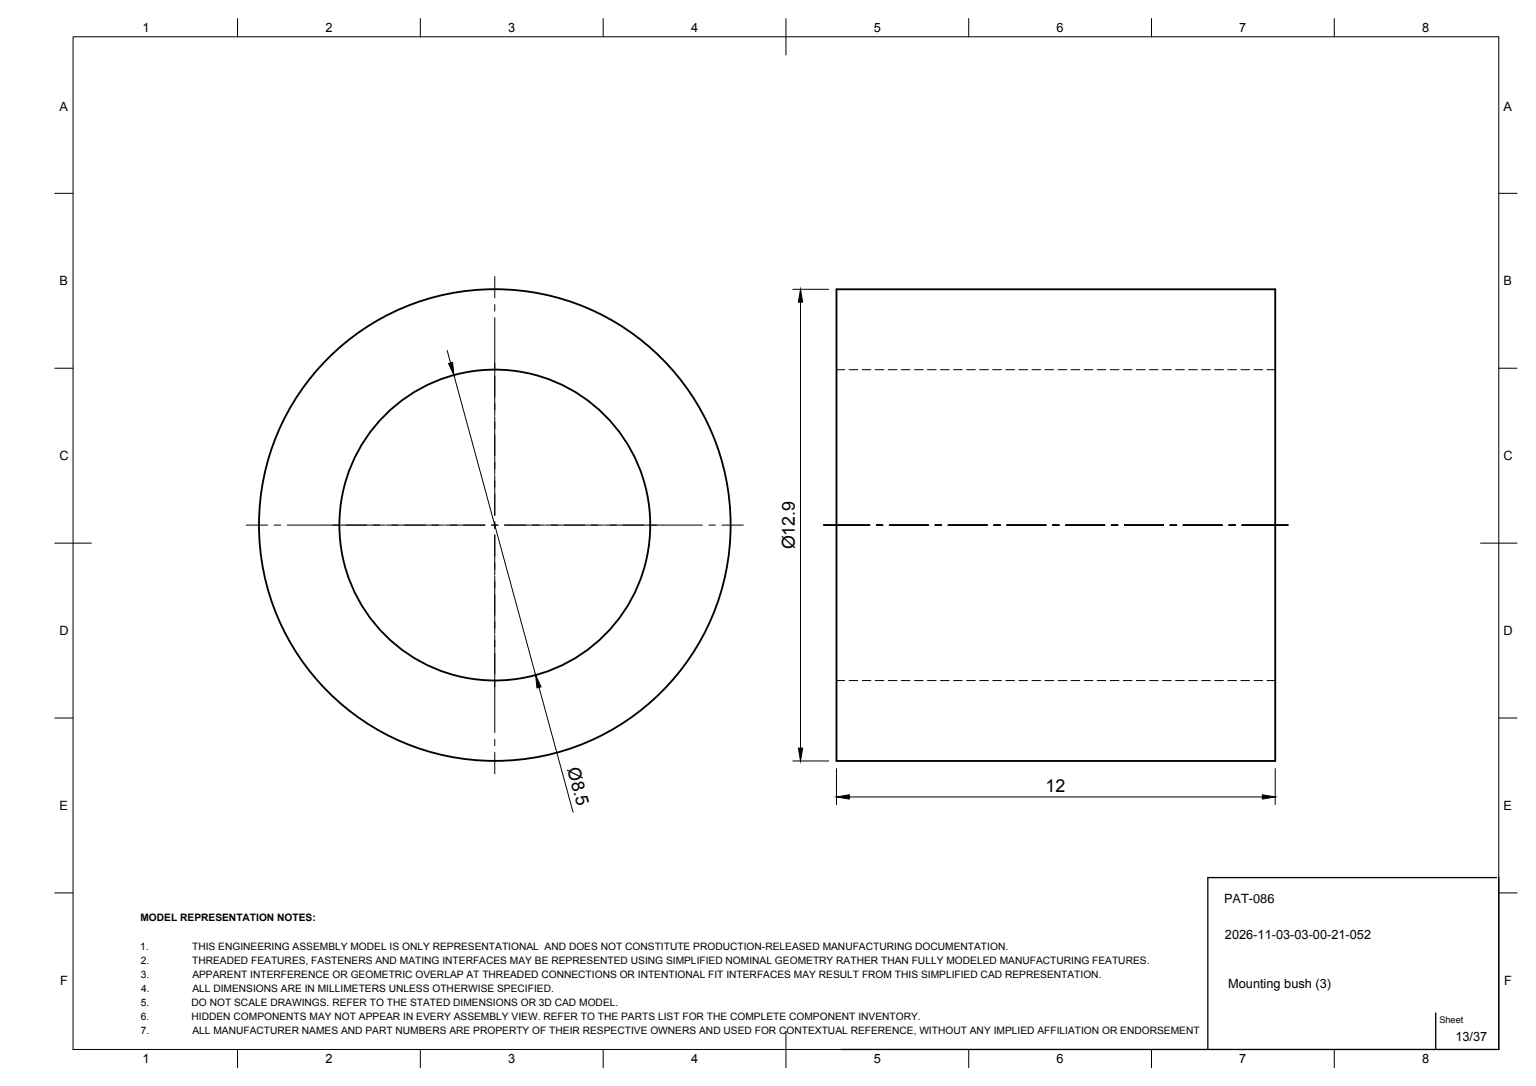
ISO-10303-21;
HEADER;
/* Generated by software containing ST-Developer
 * from STEP Tools, Inc. (www.steptools.com) 
 */

FILE_DESCRIPTION(
/* description */ ('Ratchet and pawl hand winch drum'),
/* implementation_level */ '2;1');

FILE_NAME(
/* name */ 'Mounting bush (3).step',
/* time_stamp */ '2026-10-27T12:42:58-07:00',
/* author */ (''),
/* organization */ (''),
/* preprocessor_version */ 'ST-DEVELOPER v20.2',
/* originating_system */ 'Autodesk Translation Framework v15.17.0.0',
/* authorisation */ '');

FILE_SCHEMA (('AUTOMOTIVE_DESIGN { 1 0 10303 214 3 1 1 }'));
ENDSEC;

DATA;
#10=MECHANICAL_DESIGN_GEOMETRIC_PRESENTATION_REPRESENTATION('',(#397),#11801);
#329=SHAPE_REPRESENTATION_RELATIONSHIP('SRR','None',#11955,#363);
#363=ADVANCED_BREP_SHAPE_REPRESENTATION('',(#432),#11772);
#397=STYLED_ITEM('',(#12206),#432);
#432=MANIFOLD_SOLID_BREP('Body1',#6274);
#514=FACE_BOUND('',#1337,.T.);
#515=FACE_BOUND('',#1339,.T.);
#645=PLANE('',#6848);
#646=PLANE('',#6849);
#920=FACE_OUTER_BOUND('',#1334,.T.);
#921=FACE_OUTER_BOUND('',#1335,.T.);
#922=FACE_OUTER_BOUND('',#1336,.T.);
#923=FACE_OUTER_BOUND('',#1338,.T.);
#1334=EDGE_LOOP('',(#4583,#4584,#4585,#4586));
#1335=EDGE_LOOP('',(#4587,#4588,#4589,#4590));
#1336=EDGE_LOOP('',(#4591));
#1337=EDGE_LOOP('',(#4592));
#1338=EDGE_LOOP('',(#4593));
#1339=EDGE_LOOP('',(#4594));
#1793=LINE('',#9602,#2304);
#1794=LINE('',#9608,#2305);
#2304=VECTOR('',#7784,0.425);
#2305=VECTOR('',#7791,0.645);
#2791=CIRCLE('',#6843,0.425);
#2792=CIRCLE('',#6844,0.425);
#2793=CIRCLE('',#6846,0.645);
#2794=CIRCLE('',#6847,0.645);
#3054=VERTEX_POINT('',#9599);
#3055=VERTEX_POINT('',#9601);
#3056=VERTEX_POINT('',#9605);
#3057=VERTEX_POINT('',#9607);
#3635=EDGE_CURVE('',#3054,#3054,#2791,.T.);
#3636=EDGE_CURVE('',#3054,#3055,#1793,.T.);
#3637=EDGE_CURVE('',#3055,#3055,#2792,.T.);
#3638=EDGE_CURVE('',#3056,#3056,#2793,.T.);
#3639=EDGE_CURVE('',#3056,#3057,#1794,.T.);
#3640=EDGE_CURVE('',#3057,#3057,#2794,.T.);
#4583=ORIENTED_EDGE('',*,*,#3635,.F.);
#4584=ORIENTED_EDGE('',*,*,#3636,.T.);
#4585=ORIENTED_EDGE('',*,*,#3637,.T.);
#4586=ORIENTED_EDGE('',*,*,#3636,.F.);
#4587=ORIENTED_EDGE('',*,*,#3638,.F.);
#4588=ORIENTED_EDGE('',*,*,#3639,.T.);
#4589=ORIENTED_EDGE('',*,*,#3640,.T.);
#4590=ORIENTED_EDGE('',*,*,#3639,.F.);
#4591=ORIENTED_EDGE('',*,*,#3638,.T.);
#4592=ORIENTED_EDGE('',*,*,#3635,.T.);
#4593=ORIENTED_EDGE('',*,*,#3640,.F.);
#4594=ORIENTED_EDGE('',*,*,#3637,.F.);
#5843=CYLINDRICAL_SURFACE('',#6842,0.425);
#5844=CYLINDRICAL_SURFACE('',#6845,0.645);
#5990=ADVANCED_FACE('',(#920),#5843,.F.);
#5991=ADVANCED_FACE('',(#921),#5844,.T.);
#5992=ADVANCED_FACE('',(#922,#514),#645,.T.);
#5993=ADVANCED_FACE('',(#923,#515),#646,.F.);
#6274=CLOSED_SHELL('',(#5990,#5991,#5992,#5993));
#6841=AXIS2_PLACEMENT_3D('',#9597,#7778,#7779);
#6842=AXIS2_PLACEMENT_3D('',#9598,#7780,#7781);
#6843=AXIS2_PLACEMENT_3D('',#9600,#7782,#7783);
#6844=AXIS2_PLACEMENT_3D('',#9603,#7785,#7786);
#6845=AXIS2_PLACEMENT_3D('',#9604,#7787,#7788);
#6846=AXIS2_PLACEMENT_3D('',#9606,#7789,#7790);
#6847=AXIS2_PLACEMENT_3D('',#9609,#7792,#7793);
#6848=AXIS2_PLACEMENT_3D('',#9610,#7794,#7795);
#6849=AXIS2_PLACEMENT_3D('',#9611,#7796,#7797);
#7778=DIRECTION('axis',(0.,0.,1.));
#7779=DIRECTION('refdir',(1.,0.,0.));
#7780=DIRECTION('center_axis',(0.,0.,1.));
#7781=DIRECTION('ref_axis',(1.,0.,0.));
#7782=DIRECTION('center_axis',(0.,0.,-1.));
#7783=DIRECTION('ref_axis',(1.,0.,0.));
#7784=DIRECTION('',(0.,0.,-1.));
#7785=DIRECTION('center_axis',(0.,0.,-1.));
#7786=DIRECTION('ref_axis',(1.,0.,0.));
#7787=DIRECTION('center_axis',(0.,0.,1.));
#7788=DIRECTION('ref_axis',(1.,0.,0.));
#7789=DIRECTION('center_axis',(0.,0.,1.));
#7790=DIRECTION('ref_axis',(1.,0.,0.));
#7791=DIRECTION('',(0.,0.,-1.));
#7792=DIRECTION('center_axis',(0.,0.,1.));
#7793=DIRECTION('ref_axis',(1.,0.,0.));
#7794=DIRECTION('center_axis',(0.,0.,1.));
#7795=DIRECTION('ref_axis',(1.,0.,0.));
#7796=DIRECTION('center_axis',(0.,0.,1.));
#7797=DIRECTION('ref_axis',(1.,0.,0.));
#9597=CARTESIAN_POINT('',(0.,0.,0.));
#9598=CARTESIAN_POINT('Origin',(4.75,16.,3.2));
#9599=CARTESIAN_POINT('',(4.325,16.,4.4));
#9600=CARTESIAN_POINT('Origin',(4.75,16.,4.4));
#9601=CARTESIAN_POINT('',(4.325,16.,3.2));
#9602=CARTESIAN_POINT('',(4.325,16.,3.2));
#9603=CARTESIAN_POINT('Origin',(4.75,16.,3.2));
#9604=CARTESIAN_POINT('Origin',(4.75,16.,3.2));
#9605=CARTESIAN_POINT('',(4.105,16.,4.4));
#9606=CARTESIAN_POINT('Origin',(4.75,16.,4.4));
#9607=CARTESIAN_POINT('',(4.105,16.,3.2));
#9608=CARTESIAN_POINT('',(4.105,16.,3.2));
#9609=CARTESIAN_POINT('Origin',(4.75,16.,3.2));
#9610=CARTESIAN_POINT('Origin',(4.75,16.,4.4));
#9611=CARTESIAN_POINT('Origin',(4.75,16.,3.2));
#11732=UNCERTAINTY_MEASURE_WITH_UNIT(LENGTH_MEASURE(0.001),#11802,
'DISTANCE_ACCURACY_VALUE',
'Maximum model space distance between geometric entities at asserted c
onnectivities');
#11761=UNCERTAINTY_MEASURE_WITH_UNIT(LENGTH_MEASURE(0.001),#11802,
'DISTANCE_ACCURACY_VALUE',
'Maximum model space distance between geometric entities at asserted c
onnectivities');
#11772=(
GEOMETRIC_REPRESENTATION_CONTEXT(3)
GLOBAL_UNCERTAINTY_ASSIGNED_CONTEXT((#11732))
GLOBAL_UNIT_ASSIGNED_CONTEXT((#11802,#11804,#11805))
REPRESENTATION_CONTEXT('','3D')
);
#11801=(
GEOMETRIC_REPRESENTATION_CONTEXT(3)
GLOBAL_UNCERTAINTY_ASSIGNED_CONTEXT((#11761))
GLOBAL_UNIT_ASSIGNED_CONTEXT((#11802,#11804,#11805))
REPRESENTATION_CONTEXT('','3D')
);
#11802=(
LENGTH_UNIT()
NAMED_UNIT(*)
SI_UNIT(.CENTI.,.METRE.)
);
#11804=(
NAMED_UNIT(*)
PLANE_ANGLE_UNIT()
SI_UNIT($,.RADIAN.)
);
#11805=(
NAMED_UNIT(*)
SI_UNIT($,.STERADIAN.)
SOLID_ANGLE_UNIT()
);
#11816=SHAPE_DEFINITION_REPRESENTATION(#11855,#11955);
#11855=PRODUCT_DEFINITION_SHAPE('',$,#11995);
#11955=SHAPE_REPRESENTATION('',(#6841),#11772);
#11984=PRODUCT_DEFINITION_CONTEXT('part definition',#12103,'design');
#11995=PRODUCT_DEFINITION('Mounting bush (3)','Mounting bush (3)',#12034,
#11984);
#12034=PRODUCT_DEFINITION_FORMATION('',$,#12115);
#12103=APPLICATION_CONTEXT(
'Core Data for Automotive Mechanical Design Process');
#12104=PRODUCT_CONTEXT('part definition',#12103,'mechanical');
#12115=PRODUCT('Mounting bush (3)','Mounting bush (3)','Mounting bush (3)',(#12104));
#12200=COLOUR_RGB('Sky Blue',0.24,0.69,0.87);
#12201=FILL_AREA_STYLE_COLOUR('',#12200);
#12202=FILL_AREA_STYLE('',(#12201));
#12203=SURFACE_STYLE_FILL_AREA(#12202);
#12204=SURFACE_SIDE_STYLE('',(#12203));
#12205=SURFACE_STYLE_USAGE(.BOTH.,#12204);
#12206=PRESENTATION_STYLE_ASSIGNMENT((#12205));
ENDSEC;
END-ISO-10303-21;
